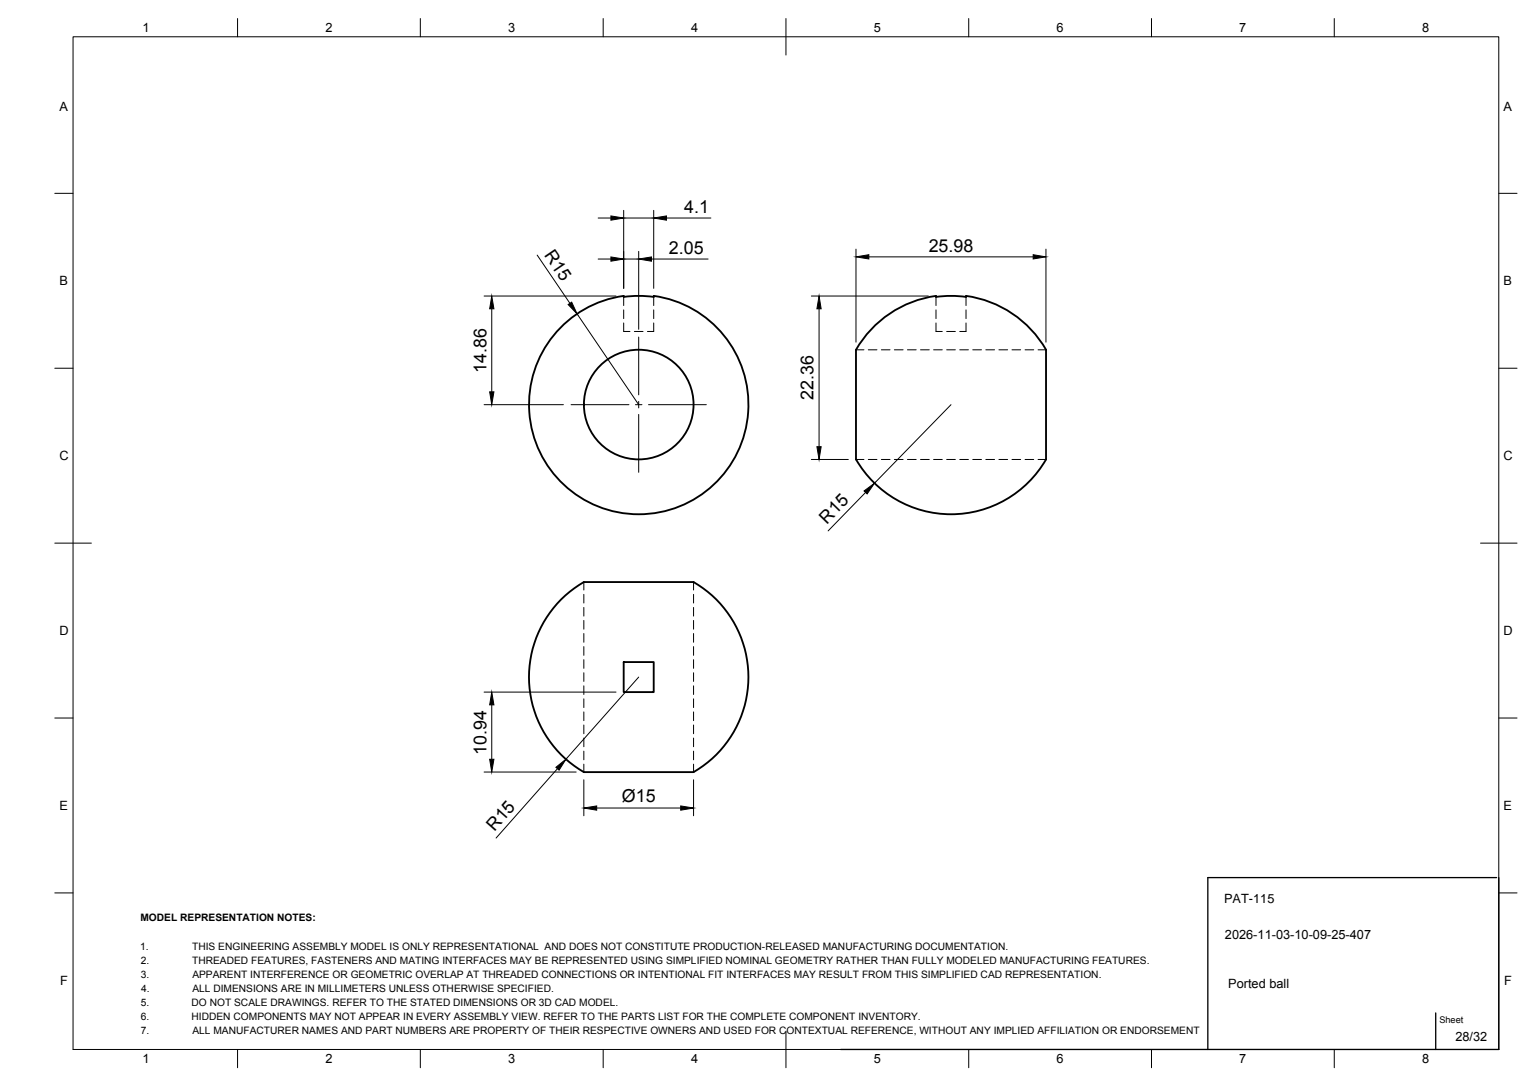
ISO-10303-21;
HEADER;
/* Generated by software containing ST-Developer
 * from STEP Tools, Inc. (www.steptools.com) 
 */

FILE_DESCRIPTION(
/* description */ ('Union bypass pipe loop'),
/* implementation_level */ '2;1');

FILE_NAME(
/* name */ 'Ported ball.step',
/* time_stamp */ '2026-10-27T21:00:29-07:00',
/* author */ (''),
/* organization */ (''),
/* preprocessor_version */ 'ST-DEVELOPER v20.2',
/* originating_system */ 'Autodesk Translation Framework v15.17.0.0',
/* authorisation */ '');

FILE_SCHEMA (('AUTOMOTIVE_DESIGN { 1 0 10303 214 3 1 1 }'));
ENDSEC;

DATA;
#10=MECHANICAL_DESIGN_GEOMETRIC_PRESENTATION_REPRESENTATION('',(#471),#10095);
#407=SHAPE_REPRESENTATION_RELATIONSHIP('SRR','None',#10277,#439);
#439=ADVANCED_BREP_SHAPE_REPRESENTATION('',(#500),#10089);
#471=STYLED_ITEM('',(#10486),#500);
#500=MANIFOLD_SOLID_BREP('Body1',#5545);
#510=SPHERICAL_SURFACE('',#6523,1.5);
#626=FACE_BOUND('',#1556,.T.);
#627=FACE_BOUND('',#1557,.T.);
#781=PLANE('',#6510);
#782=PLANE('',#6512);
#783=PLANE('',#6515);
#784=PLANE('',#6517);
#785=PLANE('',#6519);
#1102=FACE_OUTER_BOUND('',#1549,.T.);
#1103=FACE_OUTER_BOUND('',#1550,.T.);
#1104=FACE_OUTER_BOUND('',#1551,.T.);
#1105=FACE_OUTER_BOUND('',#1552,.T.);
#1106=FACE_OUTER_BOUND('',#1553,.T.);
#1107=FACE_OUTER_BOUND('',#1554,.T.);
#1108=FACE_OUTER_BOUND('',#1555,.T.);
#1549=EDGE_LOOP('',(#4810,#4811,#4812,#4813));
#1550=EDGE_LOOP('',(#4814,#4815,#4816,#4817,#4818));
#1551=EDGE_LOOP('',(#4819,#4820,#4821,#4822));
#1552=EDGE_LOOP('',(#4823,#4824,#4825,#4826));
#1553=EDGE_LOOP('',(#4827,#4828,#4829,#4830));
#1554=EDGE_LOOP('',(#4831,#4832,#4833,#4834));
#1555=EDGE_LOOP('',(#4835,#4836,#4837,#4838,#4839,#4840,#4841));
#1556=EDGE_LOOP('',(#4842));
#1557=EDGE_LOOP('',(#4843));
#1895=LINE('',#9727,#2271);
#1896=LINE('',#9729,#2272);
#1897=LINE('',#9730,#2273);
#1898=LINE('',#9735,#2274);
#1899=LINE('',#9737,#2275);
#1900=LINE('',#9743,#2276);
#1901=LINE('',#9744,#2277);
#1902=LINE('',#9747,#2278);
#1903=LINE('',#9753,#2279);
#2271=VECTOR('',#8105,1.);
#2272=VECTOR('',#8106,1.);
#2273=VECTOR('',#8107,1.);
#2274=VECTOR('',#8112,1.);
#2275=VECTOR('',#8113,1.);
#2276=VECTOR('',#8120,1.);
#2277=VECTOR('',#8121,1.);
#2278=VECTOR('',#8126,1.);
#2279=VECTOR('',#8133,0.75);
#2599=CIRCLE('',#6511,1.48592563743951);
#2600=CIRCLE('',#6513,1.48592563743951);
#2601=CIRCLE('',#6514,1.48592563743951);
#2602=CIRCLE('',#6516,1.48592563743951);
#2603=CIRCLE('',#6518,1.48592563743951);
#2604=CIRCLE('',#6521,0.75);
#2605=CIRCLE('',#6522,0.75);
#2606=CIRCLE('',#6524,1.5);
#2980=VERTEX_POINT('',#9723);
#2981=VERTEX_POINT('',#9724);
#2982=VERTEX_POINT('',#9726);
#2983=VERTEX_POINT('',#9728);
#2984=VERTEX_POINT('',#9732);
#2985=VERTEX_POINT('',#9734);
#2986=VERTEX_POINT('',#9736);
#2987=VERTEX_POINT('',#9740);
#2988=VERTEX_POINT('',#9742);
#2989=VERTEX_POINT('',#9750);
#2990=VERTEX_POINT('',#9752);
#2991=VERTEX_POINT('',#9756);
#3603=EDGE_CURVE('',#2980,#2981,#2599,.T.);
#3604=EDGE_CURVE('',#2982,#2980,#1895,.T.);
#3605=EDGE_CURVE('',#2983,#2982,#1896,.T.);
#3606=EDGE_CURVE('',#2983,#2981,#1897,.T.);
#3607=EDGE_CURVE('',#2981,#2984,#2600,.T.);
#3608=EDGE_CURVE('',#2985,#2983,#1898,.T.);
#3609=EDGE_CURVE('',#2985,#2986,#1899,.T.);
#3610=EDGE_CURVE('',#2984,#2986,#2601,.T.);
#3611=EDGE_CURVE('',#2986,#2987,#2602,.T.);
#3612=EDGE_CURVE('',#2988,#2985,#1900,.T.);
#3613=EDGE_CURVE('',#2988,#2987,#1901,.T.);
#3614=EDGE_CURVE('',#2987,#2980,#2603,.T.);
#3615=EDGE_CURVE('',#2982,#2988,#1902,.T.);
#3616=EDGE_CURVE('',#2989,#2989,#2604,.T.);
#3617=EDGE_CURVE('',#2989,#2990,#1903,.T.);
#3618=EDGE_CURVE('',#2990,#2990,#2605,.T.);
#3619=EDGE_CURVE('',#2984,#2991,#2606,.T.);
#4810=ORIENTED_EDGE('',*,*,#3603,.F.);
#4811=ORIENTED_EDGE('',*,*,#3604,.F.);
#4812=ORIENTED_EDGE('',*,*,#3605,.F.);
#4813=ORIENTED_EDGE('',*,*,#3606,.T.);
#4814=ORIENTED_EDGE('',*,*,#3607,.F.);
#4815=ORIENTED_EDGE('',*,*,#3606,.F.);
#4816=ORIENTED_EDGE('',*,*,#3608,.F.);
#4817=ORIENTED_EDGE('',*,*,#3609,.T.);
#4818=ORIENTED_EDGE('',*,*,#3610,.F.);
#4819=ORIENTED_EDGE('',*,*,#3611,.F.);
#4820=ORIENTED_EDGE('',*,*,#3609,.F.);
#4821=ORIENTED_EDGE('',*,*,#3612,.F.);
#4822=ORIENTED_EDGE('',*,*,#3613,.T.);
#4823=ORIENTED_EDGE('',*,*,#3614,.F.);
#4824=ORIENTED_EDGE('',*,*,#3613,.F.);
#4825=ORIENTED_EDGE('',*,*,#3615,.F.);
#4826=ORIENTED_EDGE('',*,*,#3604,.T.);
#4827=ORIENTED_EDGE('',*,*,#3608,.T.);
#4828=ORIENTED_EDGE('',*,*,#3605,.T.);
#4829=ORIENTED_EDGE('',*,*,#3615,.T.);
#4830=ORIENTED_EDGE('',*,*,#3612,.T.);
#4831=ORIENTED_EDGE('',*,*,#3616,.F.);
#4832=ORIENTED_EDGE('',*,*,#3617,.T.);
#4833=ORIENTED_EDGE('',*,*,#3618,.F.);
#4834=ORIENTED_EDGE('',*,*,#3617,.F.);
#4835=ORIENTED_EDGE('',*,*,#3611,.T.);
#4836=ORIENTED_EDGE('',*,*,#3614,.T.);
#4837=ORIENTED_EDGE('',*,*,#3603,.T.);
#4838=ORIENTED_EDGE('',*,*,#3607,.T.);
#4839=ORIENTED_EDGE('',*,*,#3619,.T.);
#4840=ORIENTED_EDGE('',*,*,#3619,.F.);
#4841=ORIENTED_EDGE('',*,*,#3610,.T.);
#4842=ORIENTED_EDGE('',*,*,#3618,.T.);
#4843=ORIENTED_EDGE('',*,*,#3616,.T.);
#5177=CYLINDRICAL_SURFACE('',#6520,0.75);
#5451=ADVANCED_FACE('',(#1102),#781,.F.);
#5452=ADVANCED_FACE('',(#1103),#782,.F.);
#5453=ADVANCED_FACE('',(#1104),#783,.F.);
#5454=ADVANCED_FACE('',(#1105),#784,.F.);
#5455=ADVANCED_FACE('',(#1106),#785,.T.);
#5456=ADVANCED_FACE('',(#1107),#5177,.F.);
#5457=ADVANCED_FACE('',(#1108,#626,#627),#510,.T.);
#5545=CLOSED_SHELL('',(#5451,#5452,#5453,#5454,#5455,#5456,#5457));
#6509=AXIS2_PLACEMENT_3D('',#9721,#8099,#8100);
#6510=AXIS2_PLACEMENT_3D('',#9722,#8101,#8102);
#6511=AXIS2_PLACEMENT_3D('',#9725,#8103,#8104);
#6512=AXIS2_PLACEMENT_3D('',#9731,#8108,#8109);
#6513=AXIS2_PLACEMENT_3D('',#9733,#8110,#8111);
#6514=AXIS2_PLACEMENT_3D('',#9738,#8114,#8115);
#6515=AXIS2_PLACEMENT_3D('',#9739,#8116,#8117);
#6516=AXIS2_PLACEMENT_3D('',#9741,#8118,#8119);
#6517=AXIS2_PLACEMENT_3D('',#9745,#8122,#8123);
#6518=AXIS2_PLACEMENT_3D('',#9746,#8124,#8125);
#6519=AXIS2_PLACEMENT_3D('',#9748,#8127,#8128);
#6520=AXIS2_PLACEMENT_3D('',#9749,#8129,#8130);
#6521=AXIS2_PLACEMENT_3D('',#9751,#8131,#8132);
#6522=AXIS2_PLACEMENT_3D('',#9754,#8134,#8135);
#6523=AXIS2_PLACEMENT_3D('',#9755,#8136,#8137);
#6524=AXIS2_PLACEMENT_3D('',#9757,#8138,#8139);
#8099=DIRECTION('axis',(0.,0.,1.));
#8100=DIRECTION('refdir',(1.,0.,0.));
#8101=DIRECTION('center_axis',(0.,-1.,0.));
#8102=DIRECTION('ref_axis',(1.,0.,0.));
#8103=DIRECTION('center_axis',(0.,-1.,0.));
#8104=DIRECTION('ref_axis',(0.,0.,1.));
#8105=DIRECTION('',(0.,0.,1.));
#8106=DIRECTION('',(1.,0.,0.));
#8107=DIRECTION('',(0.,0.,1.));
#8108=DIRECTION('center_axis',(-1.,0.,0.));
#8109=DIRECTION('ref_axis',(0.,-1.,0.));
#8110=DIRECTION('center_axis',(-1.,0.,0.));
#8111=DIRECTION('ref_axis',(0.,0.,-1.));
#8112=DIRECTION('',(0.,-1.,0.));
#8113=DIRECTION('',(0.,0.,1.));
#8114=DIRECTION('center_axis',(-1.,0.,0.));
#8115=DIRECTION('ref_axis',(0.,0.,-1.));
#8116=DIRECTION('center_axis',(0.,1.,0.));
#8117=DIRECTION('ref_axis',(-1.,0.,0.));
#8118=DIRECTION('center_axis',(0.,1.,0.));
#8119=DIRECTION('ref_axis',(0.,0.,-1.));
#8120=DIRECTION('',(-1.,0.,0.));
#8121=DIRECTION('',(0.,0.,1.));
#8122=DIRECTION('center_axis',(1.,0.,0.));
#8123=DIRECTION('ref_axis',(0.,1.,0.));
#8124=DIRECTION('center_axis',(1.,0.,0.));
#8125=DIRECTION('ref_axis',(0.,0.,1.));
#8126=DIRECTION('',(0.,1.,0.));
#8127=DIRECTION('center_axis',(0.,0.,1.));
#8128=DIRECTION('ref_axis',(1.,0.,0.));
#8129=DIRECTION('center_axis',(0.,1.,0.));
#8130=DIRECTION('ref_axis',(1.,0.,0.));
#8131=DIRECTION('center_axis',(0.,1.,0.));
#8132=DIRECTION('ref_axis',(1.,0.,0.));
#8133=DIRECTION('',(0.,1.,0.));
#8134=DIRECTION('center_axis',(0.,-1.,0.));
#8135=DIRECTION('ref_axis',(1.,0.,0.));
#8136=DIRECTION('center_axis',(6.12323399573677E-17,0.,1.));
#8137=DIRECTION('ref_axis',(1.,0.,0.));
#8138=DIRECTION('center_axis',(1.22464679914735E-16,-1.,0.));
#8139=DIRECTION('ref_axis',(-1.,-1.22464679914735E-16,0.));
#9721=CARTESIAN_POINT('',(0.,0.,0.));
#9722=CARTESIAN_POINT('Origin',(-0.205,-0.205,6.));
#9723=CARTESIAN_POINT('',(0.205,-0.205,6.47171668469172));
#9724=CARTESIAN_POINT('',(-0.205,-0.205,6.47171668469172));
#9725=CARTESIAN_POINT('Origin',(0.,-0.205,5.));
#9726=CARTESIAN_POINT('',(0.205,-0.205,6.));
#9727=CARTESIAN_POINT('',(0.205,-0.205,6.));
#9728=CARTESIAN_POINT('',(-0.205,-0.205,6.));
#9729=CARTESIAN_POINT('',(-0.205,-0.205,6.));
#9730=CARTESIAN_POINT('',(-0.205,-0.205,6.));
#9731=CARTESIAN_POINT('Origin',(-0.205,0.205,6.));
#9732=CARTESIAN_POINT('',(-0.205,-2.51052593825207E-17,6.48592563743951));
#9733=CARTESIAN_POINT('Origin',(-0.205,0.,5.));
#9734=CARTESIAN_POINT('',(-0.205,0.205,6.));
#9735=CARTESIAN_POINT('',(-0.205,0.205,6.));
#9736=CARTESIAN_POINT('',(-0.205,0.205,6.47171668469172));
#9737=CARTESIAN_POINT('',(-0.205,0.205,6.));
#9738=CARTESIAN_POINT('Origin',(-0.205,0.,5.));
#9739=CARTESIAN_POINT('Origin',(0.205,0.205,6.));
#9740=CARTESIAN_POINT('',(0.205,0.205,6.47171668469172));
#9741=CARTESIAN_POINT('Origin',(0.,0.205,5.));
#9742=CARTESIAN_POINT('',(0.205,0.205,6.));
#9743=CARTESIAN_POINT('',(0.205,0.205,6.));
#9744=CARTESIAN_POINT('',(0.205,0.205,6.));
#9745=CARTESIAN_POINT('Origin',(0.205,-0.205,6.));
#9746=CARTESIAN_POINT('Origin',(0.205,0.,5.));
#9747=CARTESIAN_POINT('',(0.205,-0.205,6.));
#9748=CARTESIAN_POINT('Origin',(0.,0.,6.));
#9749=CARTESIAN_POINT('Origin',(0.,-1.6,5.));
#9750=CARTESIAN_POINT('',(-0.75,-1.29903810567666,5.));
#9751=CARTESIAN_POINT('Origin',(0.,-1.29903810567666,5.));
#9752=CARTESIAN_POINT('',(-0.75,1.29903810567666,5.));
#9753=CARTESIAN_POINT('',(-0.75,-1.6,5.));
#9754=CARTESIAN_POINT('Origin',(0.,1.29903810567666,5.));
#9755=CARTESIAN_POINT('Origin',(0.,0.,5.));
#9756=CARTESIAN_POINT('',(-9.18485099360515E-17,-1.12481983699639E-32,3.5));
#9757=CARTESIAN_POINT('Origin',(0.,0.,5.));
#10052=UNCERTAINTY_MEASURE_WITH_UNIT(LENGTH_MEASURE(0.001),#10096,
'DISTANCE_ACCURACY_VALUE',
'Maximum model space distance between geometric entities at asserted c
onnectivities');
#10058=UNCERTAINTY_MEASURE_WITH_UNIT(LENGTH_MEASURE(0.001),#10096,
'DISTANCE_ACCURACY_VALUE',
'Maximum model space distance between geometric entities at asserted c
onnectivities');
#10089=(
GEOMETRIC_REPRESENTATION_CONTEXT(3)
GLOBAL_UNCERTAINTY_ASSIGNED_CONTEXT((#10052))
GLOBAL_UNIT_ASSIGNED_CONTEXT((#10096,#10098,#10099))
REPRESENTATION_CONTEXT('','3D')
);
#10095=(
GEOMETRIC_REPRESENTATION_CONTEXT(3)
GLOBAL_UNCERTAINTY_ASSIGNED_CONTEXT((#10058))
GLOBAL_UNIT_ASSIGNED_CONTEXT((#10096,#10098,#10099))
REPRESENTATION_CONTEXT('','3D')
);
#10096=(
LENGTH_UNIT()
NAMED_UNIT(*)
SI_UNIT(.CENTI.,.METRE.)
);
#10098=(
NAMED_UNIT(*)
PLANE_ANGLE_UNIT()
SI_UNIT($,.RADIAN.)
);
#10099=(
NAMED_UNIT(*)
SI_UNIT($,.STERADIAN.)
SOLID_ANGLE_UNIT()
);
#10130=SHAPE_DEFINITION_REPRESENTATION(#10233,#10277);
#10233=PRODUCT_DEFINITION_SHAPE('',$,#10314);
#10277=SHAPE_REPRESENTATION('',(#6509),#10089);
#10283=PRODUCT_DEFINITION_CONTEXT('part definition',#10393,'design');
#10314=PRODUCT_DEFINITION('Ported ball','Ported ball',#10350,#10283);
#10350=PRODUCT_DEFINITION_FORMATION('',$,#10425);
#10393=APPLICATION_CONTEXT(
'Core Data for Automotive Mechanical Design Process');
#10394=PRODUCT_CONTEXT('part definition',#10393,'mechanical');
#10425=PRODUCT('Ported ball','Ported ball','Ported ball',(#10394));
#10480=COLOUR_RGB('Light Blue',0.38,0.62,0.78);
#10481=FILL_AREA_STYLE_COLOUR('',#10480);
#10482=FILL_AREA_STYLE('',(#10481));
#10483=SURFACE_STYLE_FILL_AREA(#10482);
#10484=SURFACE_SIDE_STYLE('',(#10483));
#10485=SURFACE_STYLE_USAGE(.BOTH.,#10484);
#10486=PRESENTATION_STYLE_ASSIGNMENT((#10485));
ENDSEC;
END-ISO-10303-21;
